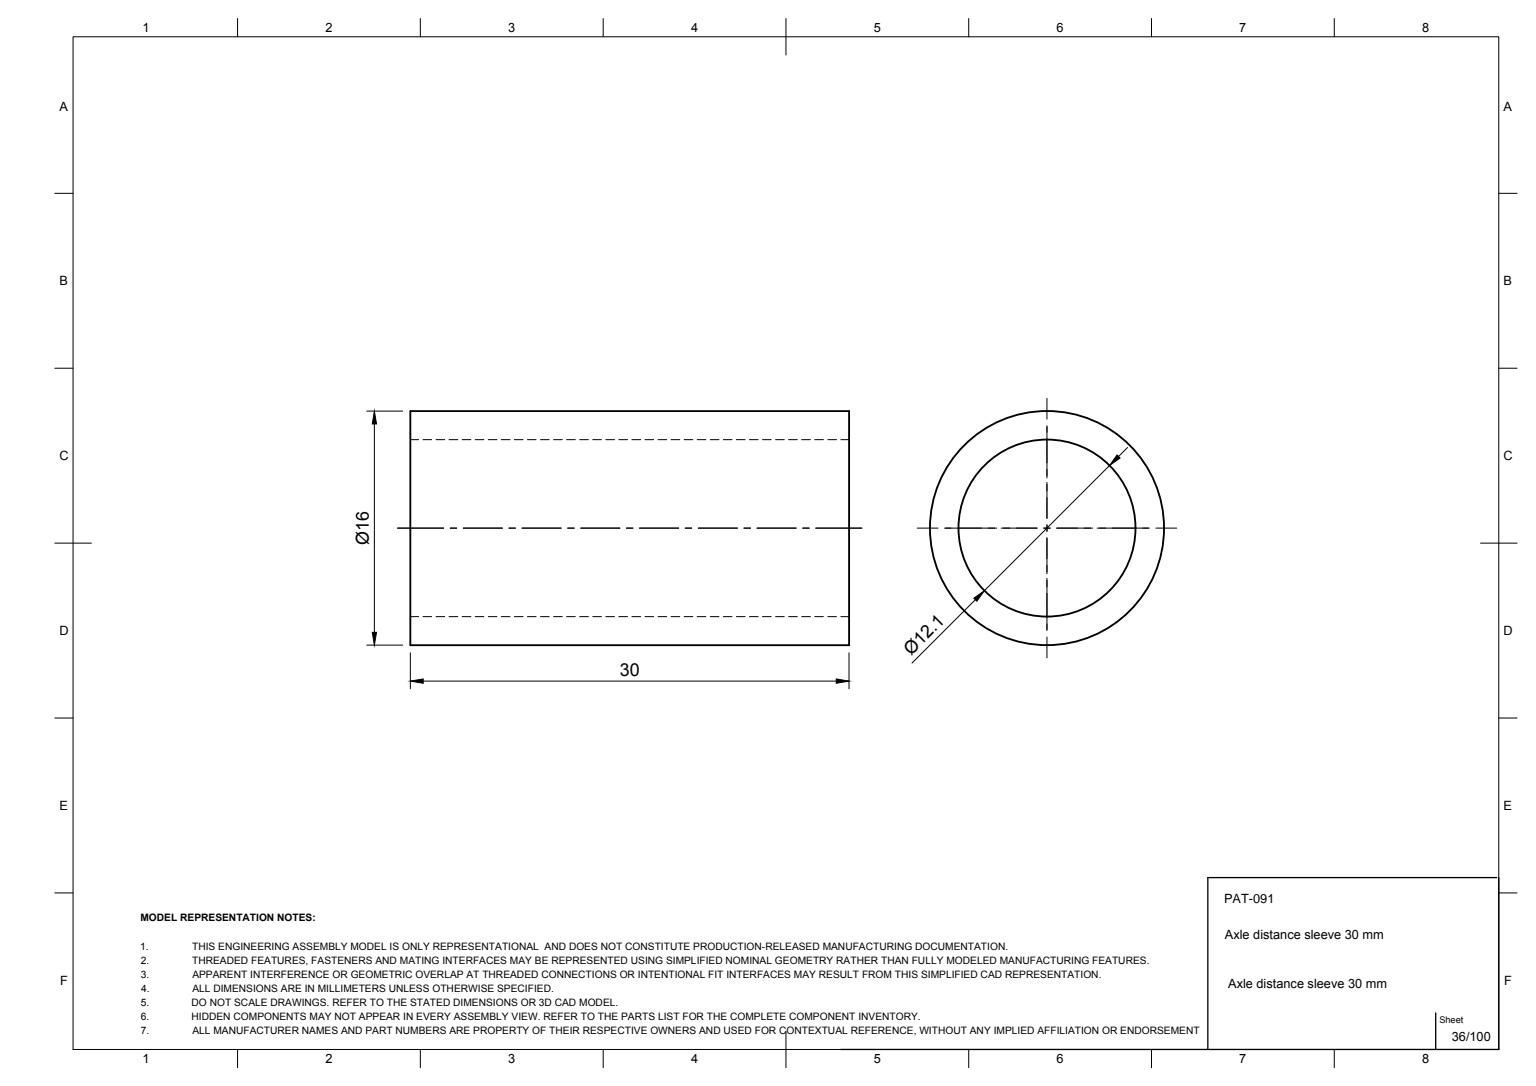
ISO-10303-21;
HEADER;
/* Generated by software containing ST-Developer
 * from STEP Tools, Inc. (www.steptools.com) 
 */

FILE_DESCRIPTION(
/* description */ ('PAT-091'),
/* implementation_level */ '2;1');

FILE_NAME(
/* name */ 'Axle distance sleeve 30 mm.step',
/* time_stamp */ '2026-10-27T15:34:44-07:00',
/* author */ (''),
/* organization */ (''),
/* preprocessor_version */ 'ST-DEVELOPER v20.2',
/* originating_system */ 'Autodesk Translation Framework v15.17.0.0',
/* authorisation */ '');

FILE_SCHEMA (('AUTOMOTIVE_DESIGN { 1 0 10303 214 3 1 1 }'));
ENDSEC;

DATA;
#10=MECHANICAL_DESIGN_GEOMETRIC_PRESENTATION_REPRESENTATION('',(#999),#25100);
#779=SHAPE_REPRESENTATION_RELATIONSHIP('SRR','None',#25541,#889);
#889=ADVANCED_BREP_SHAPE_REPRESENTATION('',(#1122),#25011);
#999=STYLED_ITEM('',(#26191),#1122);
#1122=MANIFOLD_SOLID_BREP('Body1',#13277);
#1387=FACE_BOUND('',#3291,.T.);
#1388=FACE_BOUND('',#3293,.T.);
#1762=PLANE('',#15081);
#1763=PLANE('',#15082);
#2298=FACE_OUTER_BOUND('',#3288,.T.);
#2299=FACE_OUTER_BOUND('',#3289,.T.);
#2300=FACE_OUTER_BOUND('',#3290,.T.);
#2301=FACE_OUTER_BOUND('',#3292,.T.);
#3288=EDGE_LOOP('',(#9968,#9969,#9970,#9971));
#3289=EDGE_LOOP('',(#9972,#9973,#9974,#9975));
#3290=EDGE_LOOP('',(#9976));
#3291=EDGE_LOOP('',(#9977));
#3292=EDGE_LOOP('',(#9978));
#3293=EDGE_LOOP('',(#9979));
#4399=LINE('',#22074,#5139);
#4400=LINE('',#22080,#5140);
#5139=VECTOR('',#17727,0.605);
#5140=VECTOR('',#17734,0.8);
#5827=CIRCLE('',#15076,0.605);
#5828=CIRCLE('',#15077,0.605);
#5829=CIRCLE('',#15079,0.8);
#5830=CIRCLE('',#15080,0.8);
#6714=VERTEX_POINT('',#22071);
#6715=VERTEX_POINT('',#22073);
#6716=VERTEX_POINT('',#22077);
#6717=VERTEX_POINT('',#22079);
#7919=EDGE_CURVE('',#6714,#6714,#5827,.T.);
#7920=EDGE_CURVE('',#6714,#6715,#4399,.T.);
#7921=EDGE_CURVE('',#6715,#6715,#5828,.T.);
#7922=EDGE_CURVE('',#6716,#6716,#5829,.T.);
#7923=EDGE_CURVE('',#6716,#6717,#4400,.T.);
#7924=EDGE_CURVE('',#6717,#6717,#5830,.T.);
#9968=ORIENTED_EDGE('',*,*,#7919,.F.);
#9969=ORIENTED_EDGE('',*,*,#7920,.T.);
#9970=ORIENTED_EDGE('',*,*,#7921,.T.);
#9971=ORIENTED_EDGE('',*,*,#7920,.F.);
#9972=ORIENTED_EDGE('',*,*,#7922,.F.);
#9973=ORIENTED_EDGE('',*,*,#7923,.T.);
#9974=ORIENTED_EDGE('',*,*,#7924,.T.);
#9975=ORIENTED_EDGE('',*,*,#7923,.F.);
#9976=ORIENTED_EDGE('',*,*,#7922,.T.);
#9977=ORIENTED_EDGE('',*,*,#7919,.T.);
#9978=ORIENTED_EDGE('',*,*,#7924,.F.);
#9979=ORIENTED_EDGE('',*,*,#7921,.F.);
#12184=CYLINDRICAL_SURFACE('',#15075,0.605);
#12185=CYLINDRICAL_SURFACE('',#15078,0.8);
#12665=ADVANCED_FACE('',(#2298),#12184,.F.);
#12666=ADVANCED_FACE('',(#2299),#12185,.T.);
#12667=ADVANCED_FACE('',(#2300,#1387),#1762,.T.);
#12668=ADVANCED_FACE('',(#2301,#1388),#1763,.F.);
#13277=CLOSED_SHELL('',(#12665,#12666,#12667,#12668));
#15074=AXIS2_PLACEMENT_3D('',#22069,#17721,#17722);
#15075=AXIS2_PLACEMENT_3D('',#22070,#17723,#17724);
#15076=AXIS2_PLACEMENT_3D('',#22072,#17725,#17726);
#15077=AXIS2_PLACEMENT_3D('',#22075,#17728,#17729);
#15078=AXIS2_PLACEMENT_3D('',#22076,#17730,#17731);
#15079=AXIS2_PLACEMENT_3D('',#22078,#17732,#17733);
#15080=AXIS2_PLACEMENT_3D('',#22081,#17735,#17736);
#15081=AXIS2_PLACEMENT_3D('',#22082,#17737,#17738);
#15082=AXIS2_PLACEMENT_3D('',#22083,#17739,#17740);
#17721=DIRECTION('axis',(0.,0.,1.));
#17722=DIRECTION('refdir',(1.,0.,0.));
#17723=DIRECTION('center_axis',(0.,1.,0.));
#17724=DIRECTION('ref_axis',(1.,0.,0.));
#17725=DIRECTION('center_axis',(0.,-1.,0.));
#17726=DIRECTION('ref_axis',(1.,0.,0.));
#17727=DIRECTION('',(0.,-1.,0.));
#17728=DIRECTION('center_axis',(0.,-1.,0.));
#17729=DIRECTION('ref_axis',(1.,0.,0.));
#17730=DIRECTION('center_axis',(0.,1.,0.));
#17731=DIRECTION('ref_axis',(1.,0.,0.));
#17732=DIRECTION('center_axis',(0.,1.,0.));
#17733=DIRECTION('ref_axis',(1.,0.,0.));
#17734=DIRECTION('',(0.,-1.,0.));
#17735=DIRECTION('center_axis',(0.,1.,0.));
#17736=DIRECTION('ref_axis',(1.,0.,0.));
#17737=DIRECTION('center_axis',(0.,1.,0.));
#17738=DIRECTION('ref_axis',(1.,0.,0.));
#17739=DIRECTION('center_axis',(0.,1.,0.));
#17740=DIRECTION('ref_axis',(1.,0.,0.));
#22069=CARTESIAN_POINT('',(0.,0.,0.));
#22070=CARTESIAN_POINT('Origin',(0.,4.,13.));
#22071=CARTESIAN_POINT('',(-0.605,7.,13.));
#22072=CARTESIAN_POINT('Origin',(0.,7.,13.));
#22073=CARTESIAN_POINT('',(-0.605,4.,13.));
#22074=CARTESIAN_POINT('',(-0.605,4.,13.));
#22075=CARTESIAN_POINT('Origin',(0.,4.,13.));
#22076=CARTESIAN_POINT('Origin',(0.,4.,13.));
#22077=CARTESIAN_POINT('',(-0.8,7.,13.));
#22078=CARTESIAN_POINT('Origin',(0.,7.,13.));
#22079=CARTESIAN_POINT('',(-0.8,4.,13.));
#22080=CARTESIAN_POINT('',(-0.8,4.,13.));
#22081=CARTESIAN_POINT('Origin',(0.,4.,13.));
#22082=CARTESIAN_POINT('Origin',(0.,7.,13.));
#22083=CARTESIAN_POINT('Origin',(0.,4.,13.));
#24890=UNCERTAINTY_MEASURE_WITH_UNIT(LENGTH_MEASURE(0.001),#25101,
'DISTANCE_ACCURACY_VALUE',
'Maximum model space distance between geometric entities at asserted c
onnectivities');
#24979=UNCERTAINTY_MEASURE_WITH_UNIT(LENGTH_MEASURE(0.001),#25101,
'DISTANCE_ACCURACY_VALUE',
'Maximum model space distance between geometric entities at asserted c
onnectivities');
#25011=(
GEOMETRIC_REPRESENTATION_CONTEXT(3)
GLOBAL_UNCERTAINTY_ASSIGNED_CONTEXT((#24890))
GLOBAL_UNIT_ASSIGNED_CONTEXT((#25101,#25103,#25104))
REPRESENTATION_CONTEXT('','3D')
);
#25100=(
GEOMETRIC_REPRESENTATION_CONTEXT(3)
GLOBAL_UNCERTAINTY_ASSIGNED_CONTEXT((#24979))
GLOBAL_UNIT_ASSIGNED_CONTEXT((#25101,#25103,#25104))
REPRESENTATION_CONTEXT('','3D')
);
#25101=(
LENGTH_UNIT()
NAMED_UNIT(*)
SI_UNIT(.CENTI.,.METRE.)
);
#25103=(
NAMED_UNIT(*)
PLANE_ANGLE_UNIT()
SI_UNIT($,.RADIAN.)
);
#25104=(
NAMED_UNIT(*)
SI_UNIT($,.STERADIAN.)
SOLID_ANGLE_UNIT()
);
#25136=SHAPE_DEFINITION_REPRESENTATION(#25256,#25541);
#25256=PRODUCT_DEFINITION_SHAPE('',$,#25662);
#25541=SHAPE_REPRESENTATION('',(#15074),#25011);
#25630=PRODUCT_DEFINITION_CONTEXT('part definition',#25992,'design');
#25662=PRODUCT_DEFINITION('Axle distance sleeve 30 mm',
'Axle distance sleeve 30 mm',#25782,#25630);
#25782=PRODUCT_DEFINITION_FORMATION('',$,#26025);
#25992=APPLICATION_CONTEXT(
'Core Data for Automotive Mechanical Design Process');
#25993=PRODUCT_CONTEXT('part definition',#25992,'mechanical');
#26025=PRODUCT('Axle distance sleeve 30 mm',
'Axle distance sleeve 30 mm','Axle distance sleeve 30 mm',(#25993));
#26185=COLOUR_RGB('Grey',0.48,0.52,0.57);
#26186=FILL_AREA_STYLE_COLOUR('',#26185);
#26187=FILL_AREA_STYLE('',(#26186));
#26188=SURFACE_STYLE_FILL_AREA(#26187);
#26189=SURFACE_SIDE_STYLE('',(#26188));
#26190=SURFACE_STYLE_USAGE(.BOTH.,#26189);
#26191=PRESENTATION_STYLE_ASSIGNMENT((#26190));
ENDSEC;
END-ISO-10303-21;
